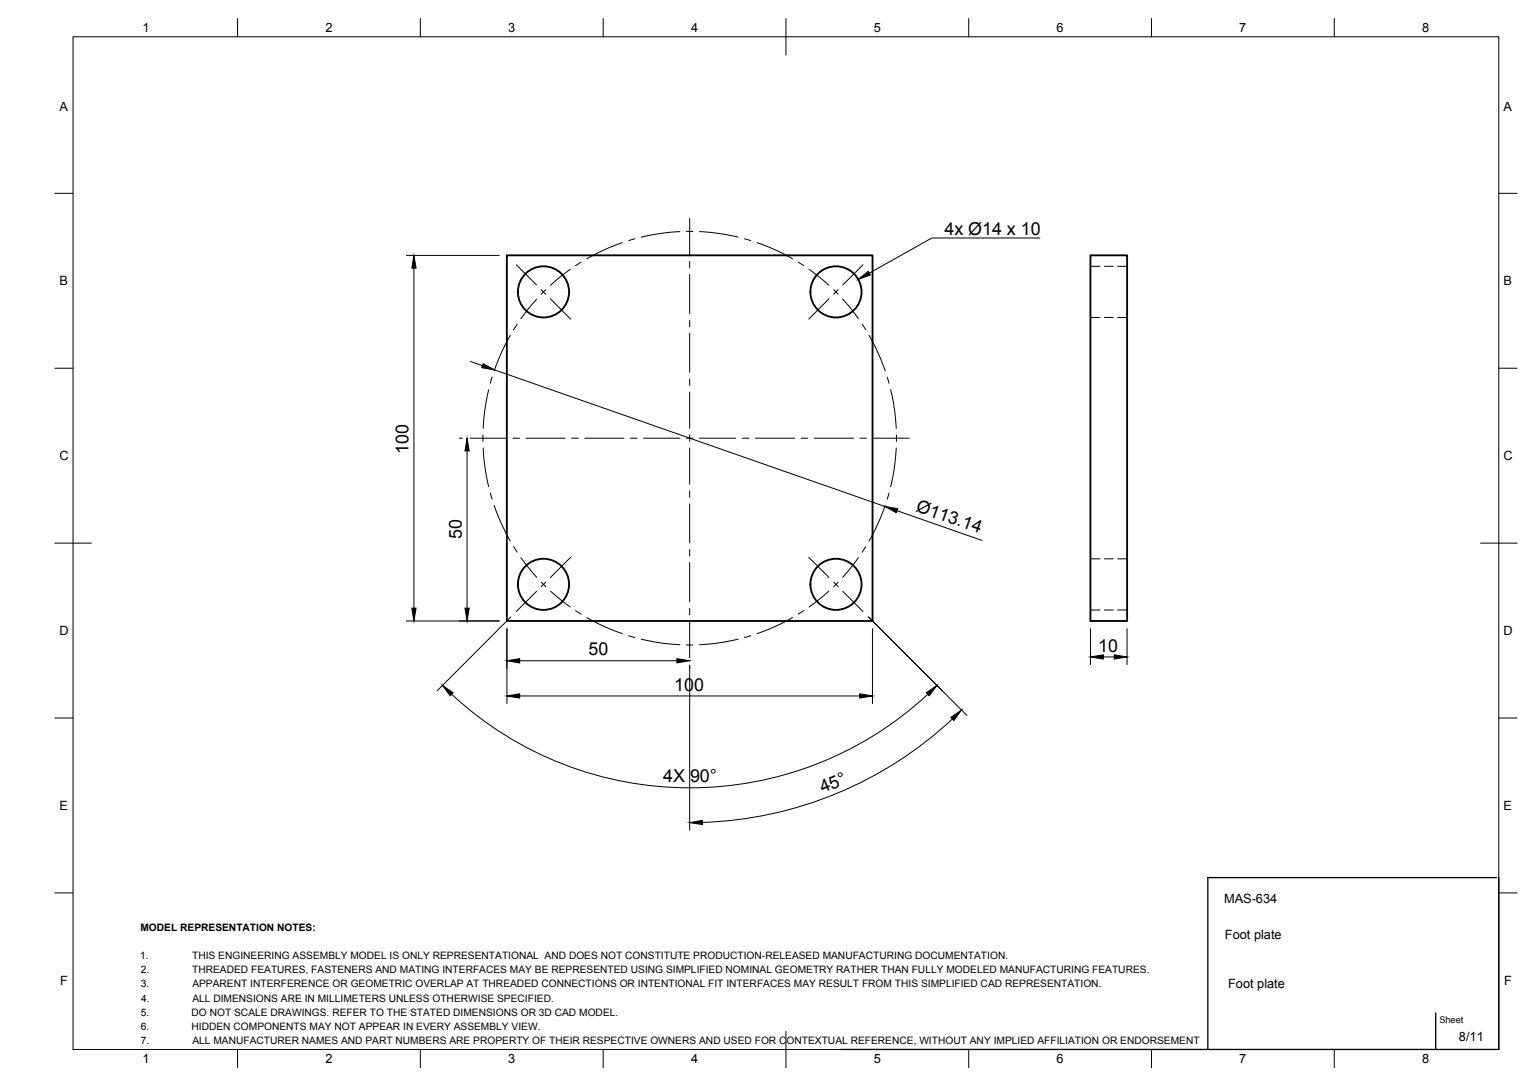
ISO-10303-21;
HEADER;
/* Generated by software containing ST-Developer
 * from STEP Tools, Inc. (www.steptools.com) 
 */

FILE_DESCRIPTION(
/* description */ ('Independent AHU equipment rack. Nominal800x600 frame on1000long40squa
re aluminum posts; two removable notched shelves; welded perimeter/cro
ss rails and rear gussets; two mounting channels; four isolation pads 
and anchor-ready feet. Imported native extrusion library retained and 
cut-length parameters customized per family. Shelf hardware uses model
ed M6 rivet nuts and screws. Weld design, floor anchors and load ratin
g require engineering selection.'),
/* implementation_level */ '2;1');

FILE_NAME(
/* name */ 'Foot plate.step',
/* time_stamp */ '2026-11-07T19:04:45-08:00',
/* author */ (''),
/* organization */ (''),
/* preprocessor_version */ 'ST-DEVELOPER v20.2',
/* originating_system */ 'Autodesk Translation Framework v15.17.0.0',
/* authorisation */ '');

FILE_SCHEMA (('AUTOMOTIVE_DESIGN { 1 0 10303 214 3 1 1 }'));
ENDSEC;

DATA;
#10=MECHANICAL_DESIGN_GEOMETRIC_PRESENTATION_REPRESENTATION('',(#340),#9777);
#318=SHAPE_REPRESENTATION_RELATIONSHIP('SRR','None',#9862,#329);
#329=ADVANCED_BREP_SHAPE_REPRESENTATION('',(#351),#9771);
#340=STYLED_ITEM('',(#9925),#351);
#351=MANIFOLD_SOLID_BREP('Body1',#3845);
#387=FACE_BOUND('',#837,.T.);
#388=FACE_BOUND('',#838,.T.);
#389=FACE_BOUND('',#839,.T.);
#390=FACE_BOUND('',#840,.T.);
#391=FACE_BOUND('',#842,.T.);
#392=FACE_BOUND('',#843,.T.);
#393=FACE_BOUND('',#844,.T.);
#394=FACE_BOUND('',#845,.T.);
#464=PLANE('',#4178);
#465=PLANE('',#4179);
#466=PLANE('',#4180);
#467=PLANE('',#4181);
#468=PLANE('',#4182);
#469=PLANE('',#4183);
#600=FACE_OUTER_BOUND('',#828,.T.);
#601=FACE_OUTER_BOUND('',#829,.T.);
#602=FACE_OUTER_BOUND('',#830,.T.);
#603=FACE_OUTER_BOUND('',#831,.T.);
#604=FACE_OUTER_BOUND('',#832,.T.);
#605=FACE_OUTER_BOUND('',#833,.T.);
#606=FACE_OUTER_BOUND('',#834,.T.);
#607=FACE_OUTER_BOUND('',#835,.T.);
#608=FACE_OUTER_BOUND('',#836,.T.);
#609=FACE_OUTER_BOUND('',#841,.T.);
#828=EDGE_LOOP('',(#3043,#3044,#3045,#3046));
#829=EDGE_LOOP('',(#3047,#3048,#3049,#3050));
#830=EDGE_LOOP('',(#3051,#3052,#3053,#3054));
#831=EDGE_LOOP('',(#3055,#3056,#3057,#3058));
#832=EDGE_LOOP('',(#3059,#3060,#3061,#3062));
#833=EDGE_LOOP('',(#3063,#3064,#3065,#3066));
#834=EDGE_LOOP('',(#3067,#3068,#3069,#3070));
#835=EDGE_LOOP('',(#3071,#3072,#3073,#3074));
#836=EDGE_LOOP('',(#3075,#3076,#3077,#3078));
#837=EDGE_LOOP('',(#3079));
#838=EDGE_LOOP('',(#3080));
#839=EDGE_LOOP('',(#3081));
#840=EDGE_LOOP('',(#3082));
#841=EDGE_LOOP('',(#3083,#3084,#3085,#3086));
#842=EDGE_LOOP('',(#3087));
#843=EDGE_LOOP('',(#3088));
#844=EDGE_LOOP('',(#3089));
#845=EDGE_LOOP('',(#3090));
#1127=LINE('',#5952,#1420);
#1128=LINE('',#5958,#1421);
#1129=LINE('',#5964,#1422);
#1130=LINE('',#5970,#1423);
#1131=LINE('',#5975,#1424);
#1132=LINE('',#5977,#1425);
#1133=LINE('',#5979,#1426);
#1134=LINE('',#5980,#1427);
#1135=LINE('',#5983,#1428);
#1136=LINE('',#5985,#1429);
#1137=LINE('',#5986,#1430);
#1138=LINE('',#5989,#1431);
#1139=LINE('',#5991,#1432);
#1140=LINE('',#5992,#1433);
#1141=LINE('',#5994,#1434);
#1142=LINE('',#5995,#1435);
#1420=VECTOR('',#4918,7.);
#1421=VECTOR('',#4925,7.);
#1422=VECTOR('',#4932,7.);
#1423=VECTOR('',#4939,7.);
#1424=VECTOR('',#4944,10.);
#1425=VECTOR('',#4945,10.);
#1426=VECTOR('',#4946,10.);
#1427=VECTOR('',#4947,10.);
#1428=VECTOR('',#4950,10.);
#1429=VECTOR('',#4951,10.);
#1430=VECTOR('',#4952,10.);
#1431=VECTOR('',#4955,10.);
#1432=VECTOR('',#4956,10.);
#1433=VECTOR('',#4957,10.);
#1434=VECTOR('',#4960,10.);
#1435=VECTOR('',#4961,10.);
#1625=CIRCLE('',#4167,7.);
#1626=CIRCLE('',#4168,7.);
#1627=CIRCLE('',#4170,7.);
#1628=CIRCLE('',#4171,7.);
#1629=CIRCLE('',#4173,7.);
#1630=CIRCLE('',#4174,7.);
#1631=CIRCLE('',#4176,7.);
#1632=CIRCLE('',#4177,7.);
#1836=VERTEX_POINT('',#5949);
#1837=VERTEX_POINT('',#5951);
#1838=VERTEX_POINT('',#5955);
#1839=VERTEX_POINT('',#5957);
#1840=VERTEX_POINT('',#5961);
#1841=VERTEX_POINT('',#5963);
#1842=VERTEX_POINT('',#5967);
#1843=VERTEX_POINT('',#5969);
#1844=VERTEX_POINT('',#5973);
#1845=VERTEX_POINT('',#5974);
#1846=VERTEX_POINT('',#5976);
#1847=VERTEX_POINT('',#5978);
#1848=VERTEX_POINT('',#5982);
#1849=VERTEX_POINT('',#5984);
#1850=VERTEX_POINT('',#5988);
#1851=VERTEX_POINT('',#5990);
#2266=EDGE_CURVE('',#1836,#1836,#1625,.T.);
#2267=EDGE_CURVE('',#1836,#1837,#1127,.T.);
#2268=EDGE_CURVE('',#1837,#1837,#1626,.T.);
#2269=EDGE_CURVE('',#1838,#1838,#1627,.T.);
#2270=EDGE_CURVE('',#1838,#1839,#1128,.T.);
#2271=EDGE_CURVE('',#1839,#1839,#1628,.T.);
#2272=EDGE_CURVE('',#1840,#1840,#1629,.T.);
#2273=EDGE_CURVE('',#1840,#1841,#1129,.T.);
#2274=EDGE_CURVE('',#1841,#1841,#1630,.T.);
#2275=EDGE_CURVE('',#1842,#1842,#1631,.T.);
#2276=EDGE_CURVE('',#1842,#1843,#1130,.T.);
#2277=EDGE_CURVE('',#1843,#1843,#1632,.T.);
#2278=EDGE_CURVE('',#1844,#1845,#1131,.T.);
#2279=EDGE_CURVE('',#1845,#1846,#1132,.T.);
#2280=EDGE_CURVE('',#1847,#1846,#1133,.T.);
#2281=EDGE_CURVE('',#1844,#1847,#1134,.T.);
#2282=EDGE_CURVE('',#1848,#1844,#1135,.T.);
#2283=EDGE_CURVE('',#1849,#1847,#1136,.T.);
#2284=EDGE_CURVE('',#1848,#1849,#1137,.T.);
#2285=EDGE_CURVE('',#1850,#1848,#1138,.T.);
#2286=EDGE_CURVE('',#1851,#1849,#1139,.T.);
#2287=EDGE_CURVE('',#1850,#1851,#1140,.T.);
#2288=EDGE_CURVE('',#1845,#1850,#1141,.T.);
#2289=EDGE_CURVE('',#1846,#1851,#1142,.T.);
#3043=ORIENTED_EDGE('',*,*,#2266,.F.);
#3044=ORIENTED_EDGE('',*,*,#2267,.T.);
#3045=ORIENTED_EDGE('',*,*,#2268,.F.);
#3046=ORIENTED_EDGE('',*,*,#2267,.F.);
#3047=ORIENTED_EDGE('',*,*,#2269,.F.);
#3048=ORIENTED_EDGE('',*,*,#2270,.T.);
#3049=ORIENTED_EDGE('',*,*,#2271,.F.);
#3050=ORIENTED_EDGE('',*,*,#2270,.F.);
#3051=ORIENTED_EDGE('',*,*,#2272,.F.);
#3052=ORIENTED_EDGE('',*,*,#2273,.T.);
#3053=ORIENTED_EDGE('',*,*,#2274,.F.);
#3054=ORIENTED_EDGE('',*,*,#2273,.F.);
#3055=ORIENTED_EDGE('',*,*,#2275,.F.);
#3056=ORIENTED_EDGE('',*,*,#2276,.T.);
#3057=ORIENTED_EDGE('',*,*,#2277,.F.);
#3058=ORIENTED_EDGE('',*,*,#2276,.F.);
#3059=ORIENTED_EDGE('',*,*,#2278,.T.);
#3060=ORIENTED_EDGE('',*,*,#2279,.T.);
#3061=ORIENTED_EDGE('',*,*,#2280,.F.);
#3062=ORIENTED_EDGE('',*,*,#2281,.F.);
#3063=ORIENTED_EDGE('',*,*,#2282,.T.);
#3064=ORIENTED_EDGE('',*,*,#2281,.T.);
#3065=ORIENTED_EDGE('',*,*,#2283,.F.);
#3066=ORIENTED_EDGE('',*,*,#2284,.F.);
#3067=ORIENTED_EDGE('',*,*,#2285,.T.);
#3068=ORIENTED_EDGE('',*,*,#2284,.T.);
#3069=ORIENTED_EDGE('',*,*,#2286,.F.);
#3070=ORIENTED_EDGE('',*,*,#2287,.F.);
#3071=ORIENTED_EDGE('',*,*,#2288,.T.);
#3072=ORIENTED_EDGE('',*,*,#2287,.T.);
#3073=ORIENTED_EDGE('',*,*,#2289,.F.);
#3074=ORIENTED_EDGE('',*,*,#2279,.F.);
#3075=ORIENTED_EDGE('',*,*,#2289,.T.);
#3076=ORIENTED_EDGE('',*,*,#2286,.T.);
#3077=ORIENTED_EDGE('',*,*,#2283,.T.);
#3078=ORIENTED_EDGE('',*,*,#2280,.T.);
#3079=ORIENTED_EDGE('',*,*,#2266,.T.);
#3080=ORIENTED_EDGE('',*,*,#2269,.T.);
#3081=ORIENTED_EDGE('',*,*,#2272,.T.);
#3082=ORIENTED_EDGE('',*,*,#2275,.T.);
#3083=ORIENTED_EDGE('',*,*,#2288,.F.);
#3084=ORIENTED_EDGE('',*,*,#2278,.F.);
#3085=ORIENTED_EDGE('',*,*,#2282,.F.);
#3086=ORIENTED_EDGE('',*,*,#2285,.F.);
#3087=ORIENTED_EDGE('',*,*,#2268,.T.);
#3088=ORIENTED_EDGE('',*,*,#2271,.T.);
#3089=ORIENTED_EDGE('',*,*,#2274,.T.);
#3090=ORIENTED_EDGE('',*,*,#2277,.T.);
#3585=CYLINDRICAL_SURFACE('',#4166,7.);
#3586=CYLINDRICAL_SURFACE('',#4169,7.);
#3587=CYLINDRICAL_SURFACE('',#4172,7.);
#3588=CYLINDRICAL_SURFACE('',#4175,7.);
#3740=ADVANCED_FACE('',(#600),#3585,.F.);
#3741=ADVANCED_FACE('',(#601),#3586,.F.);
#3742=ADVANCED_FACE('',(#602),#3587,.F.);
#3743=ADVANCED_FACE('',(#603),#3588,.F.);
#3744=ADVANCED_FACE('',(#604),#464,.T.);
#3745=ADVANCED_FACE('',(#605),#465,.T.);
#3746=ADVANCED_FACE('',(#606),#466,.T.);
#3747=ADVANCED_FACE('',(#607),#467,.T.);
#3748=ADVANCED_FACE('',(#608,#387,#388,#389,#390),#468,.T.);
#3749=ADVANCED_FACE('',(#609,#391,#392,#393,#394),#469,.F.);
#3845=CLOSED_SHELL('',(#3740,#3741,#3742,#3743,#3744,#3745,#3746,#3747,
#3748,#3749));
#4165=AXIS2_PLACEMENT_3D('',#5947,#4912,#4913);
#4166=AXIS2_PLACEMENT_3D('',#5948,#4914,#4915);
#4167=AXIS2_PLACEMENT_3D('',#5950,#4916,#4917);
#4168=AXIS2_PLACEMENT_3D('',#5953,#4919,#4920);
#4169=AXIS2_PLACEMENT_3D('',#5954,#4921,#4922);
#4170=AXIS2_PLACEMENT_3D('',#5956,#4923,#4924);
#4171=AXIS2_PLACEMENT_3D('',#5959,#4926,#4927);
#4172=AXIS2_PLACEMENT_3D('',#5960,#4928,#4929);
#4173=AXIS2_PLACEMENT_3D('',#5962,#4930,#4931);
#4174=AXIS2_PLACEMENT_3D('',#5965,#4933,#4934);
#4175=AXIS2_PLACEMENT_3D('',#5966,#4935,#4936);
#4176=AXIS2_PLACEMENT_3D('',#5968,#4937,#4938);
#4177=AXIS2_PLACEMENT_3D('',#5971,#4940,#4941);
#4178=AXIS2_PLACEMENT_3D('',#5972,#4942,#4943);
#4179=AXIS2_PLACEMENT_3D('',#5981,#4948,#4949);
#4180=AXIS2_PLACEMENT_3D('',#5987,#4953,#4954);
#4181=AXIS2_PLACEMENT_3D('',#5993,#4958,#4959);
#4182=AXIS2_PLACEMENT_3D('',#5996,#4962,#4963);
#4183=AXIS2_PLACEMENT_3D('',#5997,#4964,#4965);
#4912=DIRECTION('axis',(0.,0.,1.));
#4913=DIRECTION('refdir',(1.,0.,0.));
#4914=DIRECTION('center_axis',(0.,0.,-1.));
#4915=DIRECTION('ref_axis',(1.,0.,0.));
#4916=DIRECTION('center_axis',(0.,0.,-1.));
#4917=DIRECTION('ref_axis',(1.,0.,0.));
#4918=DIRECTION('',(0.,0.,-1.));
#4919=DIRECTION('center_axis',(0.,0.,1.));
#4920=DIRECTION('ref_axis',(1.,0.,0.));
#4921=DIRECTION('center_axis',(0.,0.,-1.));
#4922=DIRECTION('ref_axis',(1.,0.,0.));
#4923=DIRECTION('center_axis',(0.,0.,-1.));
#4924=DIRECTION('ref_axis',(1.,0.,0.));
#4925=DIRECTION('',(0.,0.,-1.));
#4926=DIRECTION('center_axis',(0.,0.,1.));
#4927=DIRECTION('ref_axis',(1.,0.,0.));
#4928=DIRECTION('center_axis',(0.,0.,-1.));
#4929=DIRECTION('ref_axis',(1.,0.,0.));
#4930=DIRECTION('center_axis',(0.,0.,-1.));
#4931=DIRECTION('ref_axis',(1.,0.,0.));
#4932=DIRECTION('',(0.,0.,-1.));
#4933=DIRECTION('center_axis',(0.,0.,1.));
#4934=DIRECTION('ref_axis',(1.,0.,0.));
#4935=DIRECTION('center_axis',(0.,0.,-1.));
#4936=DIRECTION('ref_axis',(1.,0.,0.));
#4937=DIRECTION('center_axis',(0.,0.,-1.));
#4938=DIRECTION('ref_axis',(1.,0.,0.));
#4939=DIRECTION('',(0.,0.,-1.));
#4940=DIRECTION('center_axis',(0.,0.,1.));
#4941=DIRECTION('ref_axis',(1.,0.,0.));
#4942=DIRECTION('center_axis',(0.,1.,0.));
#4943=DIRECTION('ref_axis',(-1.,0.,0.));
#4944=DIRECTION('',(-1.,0.,0.));
#4945=DIRECTION('',(0.,0.,1.));
#4946=DIRECTION('',(-1.,0.,0.));
#4947=DIRECTION('',(0.,0.,1.));
#4948=DIRECTION('center_axis',(1.,0.,0.));
#4949=DIRECTION('ref_axis',(0.,1.,0.));
#4950=DIRECTION('',(0.,1.,0.));
#4951=DIRECTION('',(0.,1.,0.));
#4952=DIRECTION('',(0.,0.,1.));
#4953=DIRECTION('center_axis',(0.,-1.,0.));
#4954=DIRECTION('ref_axis',(1.,0.,0.));
#4955=DIRECTION('',(1.,0.,0.));
#4956=DIRECTION('',(1.,0.,0.));
#4957=DIRECTION('',(0.,0.,1.));
#4958=DIRECTION('center_axis',(-1.,0.,0.));
#4959=DIRECTION('ref_axis',(0.,-1.,0.));
#4960=DIRECTION('',(0.,-1.,0.));
#4961=DIRECTION('',(0.,-1.,0.));
#4962=DIRECTION('center_axis',(0.,0.,1.));
#4963=DIRECTION('ref_axis',(1.,0.,0.));
#4964=DIRECTION('center_axis',(0.,0.,1.));
#4965=DIRECTION('ref_axis',(1.,0.,0.));
#5947=CARTESIAN_POINT('',(0.,0.,0.));
#5948=CARTESIAN_POINT('Origin',(40.,-40.,5.));
#5949=CARTESIAN_POINT('',(33.,-40.,10.));
#5950=CARTESIAN_POINT('Origin',(40.,-40.,10.));
#5951=CARTESIAN_POINT('',(33.,-40.,0.));
#5952=CARTESIAN_POINT('',(33.,-40.,5.));
#5953=CARTESIAN_POINT('Origin',(40.,-40.,0.));
#5954=CARTESIAN_POINT('Origin',(-40.,-40.,5.));
#5955=CARTESIAN_POINT('',(-47.,-40.,10.));
#5956=CARTESIAN_POINT('Origin',(-40.,-40.,10.));
#5957=CARTESIAN_POINT('',(-47.,-40.,0.));
#5958=CARTESIAN_POINT('',(-47.,-40.,5.));
#5959=CARTESIAN_POINT('Origin',(-40.,-40.,0.));
#5960=CARTESIAN_POINT('Origin',(-40.,40.,5.));
#5961=CARTESIAN_POINT('',(-47.,40.,10.));
#5962=CARTESIAN_POINT('Origin',(-40.,40.,10.));
#5963=CARTESIAN_POINT('',(-47.,40.,0.));
#5964=CARTESIAN_POINT('',(-47.,40.,5.));
#5965=CARTESIAN_POINT('Origin',(-40.,40.,0.));
#5966=CARTESIAN_POINT('Origin',(40.,40.,5.));
#5967=CARTESIAN_POINT('',(33.,40.,10.));
#5968=CARTESIAN_POINT('Origin',(40.,40.,10.));
#5969=CARTESIAN_POINT('',(33.,40.,0.));
#5970=CARTESIAN_POINT('',(33.,40.,5.));
#5971=CARTESIAN_POINT('Origin',(40.,40.,0.));
#5972=CARTESIAN_POINT('Origin',(50.,50.,0.));
#5973=CARTESIAN_POINT('',(50.,50.,0.));
#5974=CARTESIAN_POINT('',(-50.,50.,0.));
#5975=CARTESIAN_POINT('',(50.,50.,0.));
#5976=CARTESIAN_POINT('',(-50.,50.,10.));
#5977=CARTESIAN_POINT('',(-50.,50.,0.));
#5978=CARTESIAN_POINT('',(50.,50.,10.));
#5979=CARTESIAN_POINT('',(50.,50.,10.));
#5980=CARTESIAN_POINT('',(50.,50.,0.));
#5981=CARTESIAN_POINT('Origin',(50.,-50.,0.));
#5982=CARTESIAN_POINT('',(50.,-50.,0.));
#5983=CARTESIAN_POINT('',(50.,-50.,0.));
#5984=CARTESIAN_POINT('',(50.,-50.,10.));
#5985=CARTESIAN_POINT('',(50.,-50.,10.));
#5986=CARTESIAN_POINT('',(50.,-50.,0.));
#5987=CARTESIAN_POINT('Origin',(-50.,-50.,0.));
#5988=CARTESIAN_POINT('',(-50.,-50.,0.));
#5989=CARTESIAN_POINT('',(-50.,-50.,0.));
#5990=CARTESIAN_POINT('',(-50.,-50.,10.));
#5991=CARTESIAN_POINT('',(-50.,-50.,10.));
#5992=CARTESIAN_POINT('',(-50.,-50.,0.));
#5993=CARTESIAN_POINT('Origin',(-50.,50.,0.));
#5994=CARTESIAN_POINT('',(-50.,50.,0.));
#5995=CARTESIAN_POINT('',(-50.,50.,10.));
#5996=CARTESIAN_POINT('Origin',(0.,0.,10.));
#5997=CARTESIAN_POINT('Origin',(0.,0.,0.));
#9758=UNCERTAINTY_MEASURE_WITH_UNIT(LENGTH_MEASURE(0.01),#9778,
'DISTANCE_ACCURACY_VALUE',
'Maximum model space distance between geometric entities at asserted c
onnectivities');
#9764=UNCERTAINTY_MEASURE_WITH_UNIT(LENGTH_MEASURE(0.01),#9778,
'DISTANCE_ACCURACY_VALUE',
'Maximum model space distance between geometric entities at asserted c
onnectivities');
#9771=(
GEOMETRIC_REPRESENTATION_CONTEXT(3)
GLOBAL_UNCERTAINTY_ASSIGNED_CONTEXT((#9758))
GLOBAL_UNIT_ASSIGNED_CONTEXT((#9778,#9780,#9781))
REPRESENTATION_CONTEXT('','3D')
);
#9777=(
GEOMETRIC_REPRESENTATION_CONTEXT(3)
GLOBAL_UNCERTAINTY_ASSIGNED_CONTEXT((#9764))
GLOBAL_UNIT_ASSIGNED_CONTEXT((#9778,#9780,#9781))
REPRESENTATION_CONTEXT('','3D')
);
#9778=(
LENGTH_UNIT()
NAMED_UNIT(*)
SI_UNIT(.MILLI.,.METRE.)
);
#9780=(
NAMED_UNIT(*)
PLANE_ANGLE_UNIT()
SI_UNIT($,.RADIAN.)
);
#9781=(
NAMED_UNIT(*)
SI_UNIT($,.STERADIAN.)
SOLID_ANGLE_UNIT()
);
#9788=SHAPE_DEFINITION_REPRESENTATION(#9800,#9862);
#9800=PRODUCT_DEFINITION_SHAPE('',$,#9875);
#9862=SHAPE_REPRESENTATION('',(#4165),#9771);
#9868=PRODUCT_DEFINITION_CONTEXT('part definition',#9906,'design');
#9875=PRODUCT_DEFINITION('Foot plate','Foot plate',#9887,#9868);
#9887=PRODUCT_DEFINITION_FORMATION('',$,#9914);
#9906=APPLICATION_CONTEXT(
'Core Data for Automotive Mechanical Design Process');
#9907=PRODUCT_CONTEXT('part definition',#9906,'mechanical');
#9914=PRODUCT('Foot plate','Foot plate',$,(#9907));
#9925=PRESENTATION_STYLE_ASSIGNMENT((#9936));
#9936=SURFACE_STYLE_USAGE(.BOTH.,#9947);
#9947=SURFACE_SIDE_STYLE('',(#9958));
#9958=SURFACE_STYLE_FILL_AREA(#9969);
#9969=FILL_AREA_STYLE('Foot gray',(#9980));
#9980=FILL_AREA_STYLE_COLOUR('Foot gray',#9991);
#9991=COLOUR_RGB('Foot gray',0.407843137254902,0.447058823529412,0.498039215686275);
ENDSEC;
END-ISO-10303-21;
